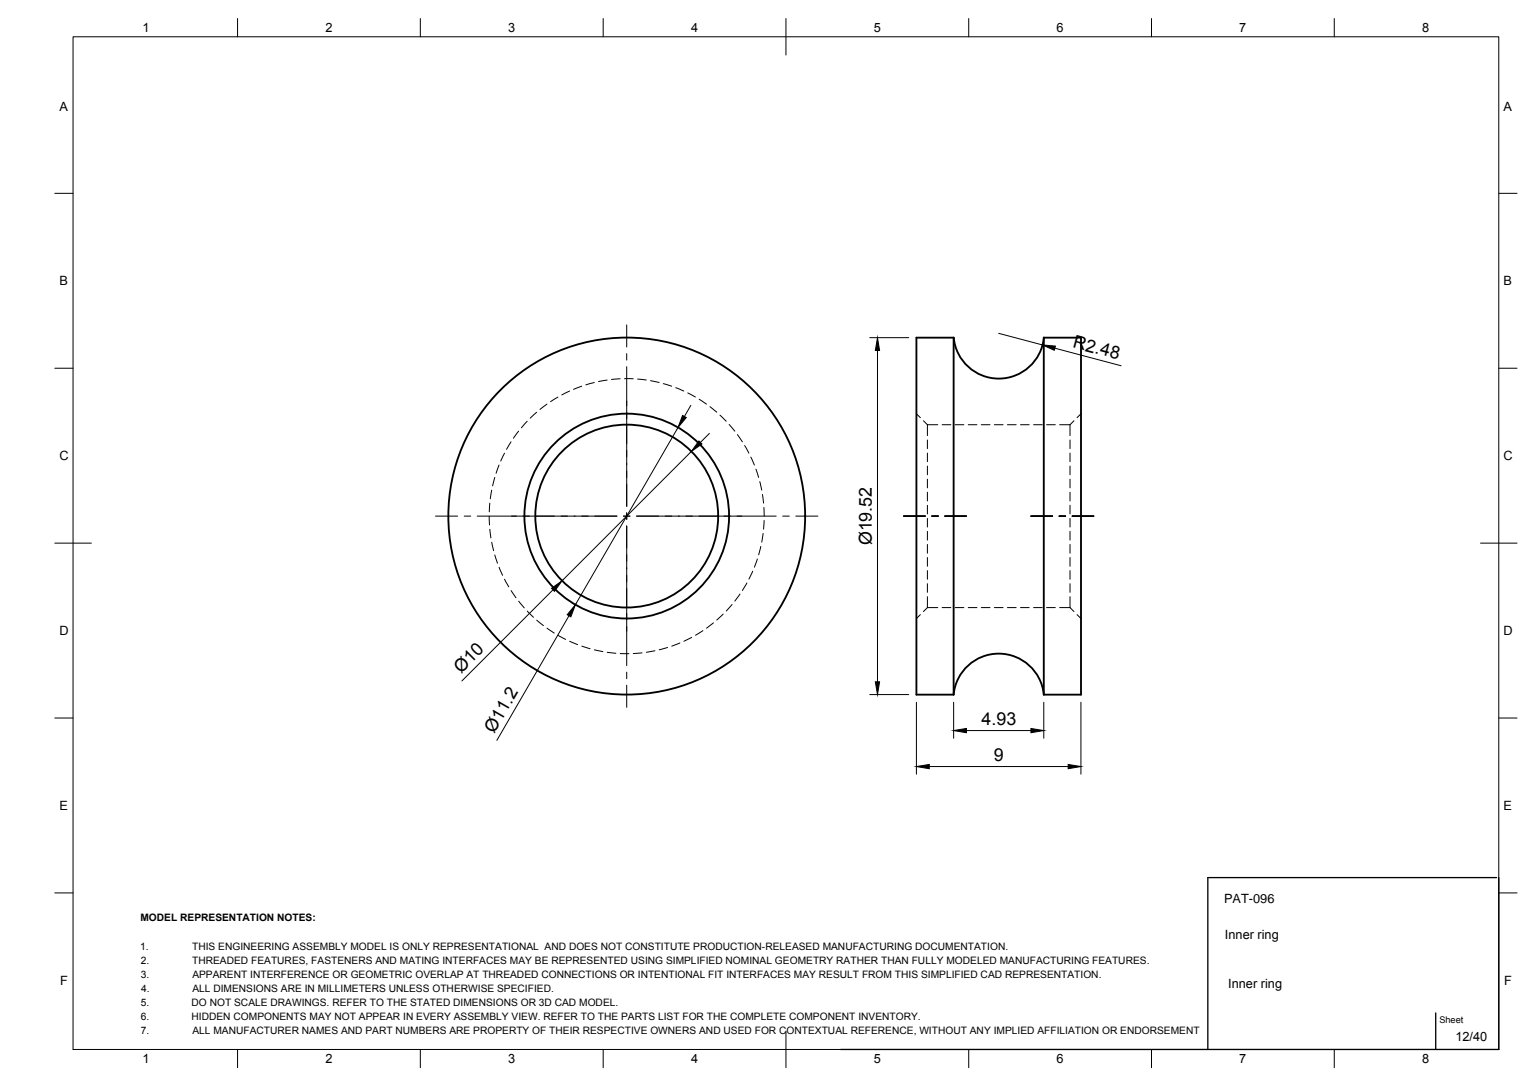
ISO-10303-21;
HEADER;
/* Generated by software containing ST-Developer
 * from STEP Tools, Inc. (www.steptools.com) 
 */

FILE_DESCRIPTION(
/* description */ ('PAT-096'),
/* implementation_level */ '2;1');

FILE_NAME(
/* name */ 'Inner ring.step',
/* time_stamp */ '2026-10-29T17:03:14-07:00',
/* author */ (''),
/* organization */ (''),
/* preprocessor_version */ 'ST-DEVELOPER v20.2',
/* originating_system */ 'Autodesk Translation Framework v15.17.0.0',
/* authorisation */ '');

FILE_SCHEMA (('AUTOMOTIVE_DESIGN { 1 0 10303 214 3 1 1 }'));
ENDSEC;

DATA;
#10=MECHANICAL_DESIGN_GEOMETRIC_PRESENTATION_REPRESENTATION('',(#402),#10650);
#279=TOROIDAL_SURFACE('',#6085,1.,0.247676);
#315=CONICAL_SURFACE('',#6096,0.53,0.785398163397448);
#316=CONICAL_SURFACE('',#6103,0.53,0.785398163397448);
#340=SHAPE_REPRESENTATION_RELATIONSHIP('SRR','None',#10801,#371);
#371=ADVANCED_BREP_SHAPE_REPRESENTATION('',(#440),#10619);
#402=STYLED_ITEM('',(#11064),#440);
#440=MANIFOLD_SOLID_BREP('Body1',#5536);
#523=FACE_BOUND('',#1258,.T.);
#524=FACE_BOUND('',#1261,.T.);
#648=PLANE('',#6098);
#649=PLANE('',#6101);
#867=FACE_OUTER_BOUND('',#1253,.T.);
#868=FACE_OUTER_BOUND('',#1254,.T.);
#869=FACE_OUTER_BOUND('',#1255,.T.);
#870=FACE_OUTER_BOUND('',#1256,.T.);
#871=FACE_OUTER_BOUND('',#1257,.T.);
#872=FACE_OUTER_BOUND('',#1259,.T.);
#873=FACE_OUTER_BOUND('',#1260,.T.);
#874=FACE_OUTER_BOUND('',#1262,.T.);
#1253=EDGE_LOOP('',(#4043,#4044,#4045,#4046,#4047,#4048));
#1254=EDGE_LOOP('',(#4049,#4050,#4051,#4052,#4053));
#1255=EDGE_LOOP('',(#4054,#4055,#4056,#4057));
#1256=EDGE_LOOP('',(#4058,#4059,#4060,#4061));
#1257=EDGE_LOOP('',(#4062));
#1258=EDGE_LOOP('',(#4063));
#1259=EDGE_LOOP('',(#4064,#4065,#4066,#4067,#4068));
#1260=EDGE_LOOP('',(#4069));
#1261=EDGE_LOOP('',(#4070));
#1262=EDGE_LOOP('',(#4071,#4072,#4073,#4074));
#1676=LINE('',#8950,#2005);
#1677=LINE('',#8956,#2006);
#1678=LINE('',#8960,#2007);
#1679=LINE('',#8966,#2008);
#1680=LINE('',#8971,#2009);
#2005=VECTOR('',#7100,0.976185);
#2006=VECTOR('',#7107,0.5);
#2007=VECTOR('',#7112,0.53);
#2008=VECTOR('',#7121,0.976185);
#2009=VECTOR('',#7128,0.53);
#2344=CIRCLE('',#6086,0.976185);
#2345=CIRCLE('',#6087,0.976185);
#2346=CIRCLE('',#6088,0.247676);
#2347=CIRCLE('',#6089,0.976185);
#2348=CIRCLE('',#6090,0.976185);
#2349=CIRCLE('',#6092,0.976185);
#2350=CIRCLE('',#6094,0.5);
#2351=CIRCLE('',#6095,0.5);
#2352=CIRCLE('',#6097,0.56);
#2353=CIRCLE('',#6100,0.976185);
#2354=CIRCLE('',#6102,0.56);
#2687=VERTEX_POINT('',#8939);
#2688=VERTEX_POINT('',#8940);
#2689=VERTEX_POINT('',#8943);
#2690=VERTEX_POINT('',#8945);
#2691=VERTEX_POINT('',#8949);
#2692=VERTEX_POINT('',#8953);
#2693=VERTEX_POINT('',#8955);
#2694=VERTEX_POINT('',#8959);
#2695=VERTEX_POINT('',#8964);
#2696=VERTEX_POINT('',#8968);
#3200=EDGE_CURVE('',#2687,#2688,#2344,.T.);
#3201=EDGE_CURVE('',#2688,#2687,#2345,.T.);
#3202=EDGE_CURVE('',#2688,#2689,#2346,.T.);
#3203=EDGE_CURVE('',#2690,#2689,#2347,.T.);
#3204=EDGE_CURVE('',#2689,#2690,#2348,.T.);
#3205=EDGE_CURVE('',#2690,#2691,#1676,.T.);
#3206=EDGE_CURVE('',#2691,#2691,#2349,.T.);
#3207=EDGE_CURVE('',#2692,#2692,#2350,.T.);
#3208=EDGE_CURVE('',#2692,#2693,#1677,.T.);
#3209=EDGE_CURVE('',#2693,#2693,#2351,.T.);
#3210=EDGE_CURVE('',#2693,#2694,#1678,.T.);
#3211=EDGE_CURVE('',#2694,#2694,#2352,.T.);
#3212=EDGE_CURVE('',#2695,#2695,#2353,.T.);
#3213=EDGE_CURVE('',#2695,#2687,#1679,.T.);
#3214=EDGE_CURVE('',#2696,#2696,#2354,.T.);
#3215=EDGE_CURVE('',#2696,#2692,#1680,.T.);
#4043=ORIENTED_EDGE('',*,*,#3200,.F.);
#4044=ORIENTED_EDGE('',*,*,#3201,.F.);
#4045=ORIENTED_EDGE('',*,*,#3202,.T.);
#4046=ORIENTED_EDGE('',*,*,#3203,.F.);
#4047=ORIENTED_EDGE('',*,*,#3204,.F.);
#4048=ORIENTED_EDGE('',*,*,#3202,.F.);
#4049=ORIENTED_EDGE('',*,*,#3203,.T.);
#4050=ORIENTED_EDGE('',*,*,#3204,.T.);
#4051=ORIENTED_EDGE('',*,*,#3205,.T.);
#4052=ORIENTED_EDGE('',*,*,#3206,.T.);
#4053=ORIENTED_EDGE('',*,*,#3205,.F.);
#4054=ORIENTED_EDGE('',*,*,#3207,.T.);
#4055=ORIENTED_EDGE('',*,*,#3208,.T.);
#4056=ORIENTED_EDGE('',*,*,#3209,.F.);
#4057=ORIENTED_EDGE('',*,*,#3208,.F.);
#4058=ORIENTED_EDGE('',*,*,#3209,.T.);
#4059=ORIENTED_EDGE('',*,*,#3210,.T.);
#4060=ORIENTED_EDGE('',*,*,#3211,.F.);
#4061=ORIENTED_EDGE('',*,*,#3210,.F.);
#4062=ORIENTED_EDGE('',*,*,#3206,.F.);
#4063=ORIENTED_EDGE('',*,*,#3211,.T.);
#4064=ORIENTED_EDGE('',*,*,#3212,.F.);
#4065=ORIENTED_EDGE('',*,*,#3213,.T.);
#4066=ORIENTED_EDGE('',*,*,#3200,.T.);
#4067=ORIENTED_EDGE('',*,*,#3201,.T.);
#4068=ORIENTED_EDGE('',*,*,#3213,.F.);
#4069=ORIENTED_EDGE('',*,*,#3212,.T.);
#4070=ORIENTED_EDGE('',*,*,#3214,.F.);
#4071=ORIENTED_EDGE('',*,*,#3214,.T.);
#4072=ORIENTED_EDGE('',*,*,#3215,.T.);
#4073=ORIENTED_EDGE('',*,*,#3207,.F.);
#4074=ORIENTED_EDGE('',*,*,#3215,.F.);
#5111=CYLINDRICAL_SURFACE('',#6091,0.976185);
#5112=CYLINDRICAL_SURFACE('',#6093,0.5);
#5113=CYLINDRICAL_SURFACE('',#6099,0.976185);
#5272=ADVANCED_FACE('',(#867),#279,.F.);
#5273=ADVANCED_FACE('',(#868),#5111,.T.);
#5274=ADVANCED_FACE('',(#869),#5112,.F.);
#5275=ADVANCED_FACE('',(#870),#315,.F.);
#5276=ADVANCED_FACE('',(#871,#523),#648,.T.);
#5277=ADVANCED_FACE('',(#872),#5113,.T.);
#5278=ADVANCED_FACE('',(#873,#524),#649,.T.);
#5279=ADVANCED_FACE('',(#874),#316,.F.);
#5536=CLOSED_SHELL('',(#5272,#5273,#5274,#5275,#5276,#5277,#5278,#5279));
#6084=AXIS2_PLACEMENT_3D('',#8937,#7084,#7085);
#6085=AXIS2_PLACEMENT_3D('',#8938,#7086,#7087);
#6086=AXIS2_PLACEMENT_3D('',#8941,#7088,#7089);
#6087=AXIS2_PLACEMENT_3D('',#8942,#7090,#7091);
#6088=AXIS2_PLACEMENT_3D('',#8944,#7092,#7093);
#6089=AXIS2_PLACEMENT_3D('',#8946,#7094,#7095);
#6090=AXIS2_PLACEMENT_3D('',#8947,#7096,#7097);
#6091=AXIS2_PLACEMENT_3D('',#8948,#7098,#7099);
#6092=AXIS2_PLACEMENT_3D('',#8951,#7101,#7102);
#6093=AXIS2_PLACEMENT_3D('',#8952,#7103,#7104);
#6094=AXIS2_PLACEMENT_3D('',#8954,#7105,#7106);
#6095=AXIS2_PLACEMENT_3D('',#8957,#7108,#7109);
#6096=AXIS2_PLACEMENT_3D('',#8958,#7110,#7111);
#6097=AXIS2_PLACEMENT_3D('',#8961,#7113,#7114);
#6098=AXIS2_PLACEMENT_3D('',#8962,#7115,#7116);
#6099=AXIS2_PLACEMENT_3D('',#8963,#7117,#7118);
#6100=AXIS2_PLACEMENT_3D('',#8965,#7119,#7120);
#6101=AXIS2_PLACEMENT_3D('',#8967,#7122,#7123);
#6102=AXIS2_PLACEMENT_3D('',#8969,#7124,#7125);
#6103=AXIS2_PLACEMENT_3D('',#8970,#7126,#7127);
#7084=DIRECTION('axis',(0.,0.,1.));
#7085=DIRECTION('refdir',(1.,0.,0.));
#7086=DIRECTION('center_axis',(0.,-1.,0.));
#7087=DIRECTION('ref_axis',(0.,0.,-1.));
#7088=DIRECTION('center_axis',(0.,-1.,0.));
#7089=DIRECTION('ref_axis',(1.,0.,0.));
#7090=DIRECTION('center_axis',(0.,-1.,0.));
#7091=DIRECTION('ref_axis',(1.,0.,0.));
#7092=DIRECTION('center_axis',(1.,0.,1.22464679914735E-16));
#7093=DIRECTION('ref_axis',(-1.22464679914735E-16,0.,1.));
#7094=DIRECTION('center_axis',(0.,1.,0.));
#7095=DIRECTION('ref_axis',(1.,0.,0.));
#7096=DIRECTION('center_axis',(0.,1.,0.));
#7097=DIRECTION('ref_axis',(1.,0.,0.));
#7098=DIRECTION('center_axis',(0.,-1.,0.));
#7099=DIRECTION('ref_axis',(1.,0.,0.));
#7100=DIRECTION('',(0.,1.,0.));
#7101=DIRECTION('center_axis',(0.,-1.,0.));
#7102=DIRECTION('ref_axis',(1.,0.,0.));
#7103=DIRECTION('center_axis',(0.,-1.,0.));
#7104=DIRECTION('ref_axis',(1.,0.,0.));
#7105=DIRECTION('center_axis',(0.,-1.,0.));
#7106=DIRECTION('ref_axis',(1.,0.,0.));
#7107=DIRECTION('',(0.,1.,0.));
#7108=DIRECTION('center_axis',(0.,-1.,0.));
#7109=DIRECTION('ref_axis',(1.,0.,0.));
#7110=DIRECTION('center_axis',(0.,1.,0.));
#7111=DIRECTION('ref_axis',(1.,0.,0.));
#7112=DIRECTION('',(-0.707106781186547,0.707106781186548,-8.65956056235493E-17));
#7113=DIRECTION('center_axis',(0.,-1.,0.));
#7114=DIRECTION('ref_axis',(1.,0.,0.));
#7115=DIRECTION('center_axis',(0.,1.,0.));
#7116=DIRECTION('ref_axis',(0.,0.,1.));
#7117=DIRECTION('center_axis',(0.,-1.,0.));
#7118=DIRECTION('ref_axis',(1.,0.,0.));
#7119=DIRECTION('center_axis',(0.,-1.,0.));
#7120=DIRECTION('ref_axis',(1.,0.,0.));
#7121=DIRECTION('',(0.,1.,0.));
#7122=DIRECTION('center_axis',(0.,-1.,0.));
#7123=DIRECTION('ref_axis',(0.,0.,-1.));
#7124=DIRECTION('center_axis',(0.,-1.,0.));
#7125=DIRECTION('ref_axis',(1.,0.,0.));
#7126=DIRECTION('center_axis',(0.,-1.,0.));
#7127=DIRECTION('ref_axis',(1.,0.,0.));
#7128=DIRECTION('',(0.707106781186547,0.707106781186548,8.65956056235493E-17));
#8937=CARTESIAN_POINT('',(0.,0.,0.));
#8938=CARTESIAN_POINT('Origin',(0.,0.,0.));
#8939=CARTESIAN_POINT('',(-0.976185,-0.246528389340863,-1.19548183562566E-16));
#8940=CARTESIAN_POINT('',(-1.19548183562566E-16,-0.246528389340863,0.976185));
#8941=CARTESIAN_POINT('Origin',(0.,-0.246528389340863,0.));
#8942=CARTESIAN_POINT('Origin',(0.,-0.246528389340863,0.));
#8943=CARTESIAN_POINT('',(-1.19548183562566E-16,0.246528389340863,0.976185));
#8944=CARTESIAN_POINT('Origin',(-1.22464679914735E-16,0.,1.));
#8945=CARTESIAN_POINT('',(-0.976185,0.246528389340863,1.19548183562566E-16));
#8946=CARTESIAN_POINT('Origin',(0.,0.246528389340863,0.));
#8947=CARTESIAN_POINT('Origin',(0.,0.246528389340863,0.));
#8948=CARTESIAN_POINT('Origin',(0.,0.,0.));
#8949=CARTESIAN_POINT('',(-0.976185,0.45,-1.19548183562566E-16));
#8950=CARTESIAN_POINT('',(-0.976185,0.,-1.19548183562566E-16));
#8951=CARTESIAN_POINT('Origin',(0.,0.45,0.));
#8952=CARTESIAN_POINT('Origin',(0.,0.,0.));
#8953=CARTESIAN_POINT('',(-0.5,-0.39,-6.12323399573677E-17));
#8954=CARTESIAN_POINT('Origin',(0.,-0.39,0.));
#8955=CARTESIAN_POINT('',(-0.5,0.39,-6.12323399573677E-17));
#8956=CARTESIAN_POINT('',(-0.5,0.,-6.12323399573677E-17));
#8957=CARTESIAN_POINT('Origin',(0.,0.39,0.));
#8958=CARTESIAN_POINT('Origin',(0.,0.42,0.));
#8959=CARTESIAN_POINT('',(-0.56,0.45,-6.85802207522518E-17));
#8960=CARTESIAN_POINT('',(-0.53,0.42,-6.49062803548097E-17));
#8961=CARTESIAN_POINT('Origin',(0.,0.45,0.));
#8962=CARTESIAN_POINT('Origin',(0.976185,0.45,0.));
#8963=CARTESIAN_POINT('Origin',(0.,0.,0.));
#8964=CARTESIAN_POINT('',(-0.976185,-0.45,-1.19548183562566E-16));
#8965=CARTESIAN_POINT('Origin',(0.,-0.45,0.));
#8966=CARTESIAN_POINT('',(-0.976185,0.,-1.19548183562566E-16));
#8967=CARTESIAN_POINT('Origin',(0.56,-0.45,0.));
#8968=CARTESIAN_POINT('',(-0.56,-0.45,-6.85802207522518E-17));
#8969=CARTESIAN_POINT('Origin',(0.,-0.45,0.));
#8970=CARTESIAN_POINT('Origin',(0.,-0.42,0.));
#8971=CARTESIAN_POINT('',(-0.53,-0.42,-6.49062803548097E-17));
#10580=UNCERTAINTY_MEASURE_WITH_UNIT(LENGTH_MEASURE(0.001),#10651,
'DISTANCE_ACCURACY_VALUE',
'Maximum model space distance between geometric entities at asserted c
onnectivities');
#10611=UNCERTAINTY_MEASURE_WITH_UNIT(LENGTH_MEASURE(0.001),#10651,
'DISTANCE_ACCURACY_VALUE',
'Maximum model space distance between geometric entities at asserted c
onnectivities');
#10619=(
GEOMETRIC_REPRESENTATION_CONTEXT(3)
GLOBAL_UNCERTAINTY_ASSIGNED_CONTEXT((#10580))
GLOBAL_UNIT_ASSIGNED_CONTEXT((#10651,#10653,#10654))
REPRESENTATION_CONTEXT('','3D')
);
#10650=(
GEOMETRIC_REPRESENTATION_CONTEXT(3)
GLOBAL_UNCERTAINTY_ASSIGNED_CONTEXT((#10611))
GLOBAL_UNIT_ASSIGNED_CONTEXT((#10651,#10653,#10654))
REPRESENTATION_CONTEXT('','3D')
);
#10651=(
LENGTH_UNIT()
NAMED_UNIT(*)
SI_UNIT(.CENTI.,.METRE.)
);
#10653=(
NAMED_UNIT(*)
PLANE_ANGLE_UNIT()
SI_UNIT($,.RADIAN.)
);
#10654=(
NAMED_UNIT(*)
SI_UNIT($,.STERADIAN.)
SOLID_ANGLE_UNIT()
);
#10662=SHAPE_DEFINITION_REPRESENTATION(#10700,#10801);
#10700=PRODUCT_DEFINITION_SHAPE('',$,#10840);
#10801=SHAPE_REPRESENTATION('',(#6084),#10619);
#10832=PRODUCT_DEFINITION_CONTEXT('part definition',#10948,'design');
#10840=PRODUCT_DEFINITION('Inner ring','Inner ring',#10878,#10832);
#10878=PRODUCT_DEFINITION_FORMATION('',$,#10957);
#10948=APPLICATION_CONTEXT(
'Core Data for Automotive Mechanical Design Process');
#10949=PRODUCT_CONTEXT('part definition',#10948,'mechanical');
#10957=PRODUCT('Inner ring','Inner ring','Inner ring',(#10949));
#11058=COLOUR_RGB('Grey',0.48,0.52,0.57);
#11059=FILL_AREA_STYLE_COLOUR('',#11058);
#11060=FILL_AREA_STYLE('',(#11059));
#11061=SURFACE_STYLE_FILL_AREA(#11060);
#11062=SURFACE_SIDE_STYLE('',(#11061));
#11063=SURFACE_STYLE_USAGE(.BOTH.,#11062);
#11064=PRESENTATION_STYLE_ASSIGNMENT((#11063));
ENDSEC;
END-ISO-10303-21;
